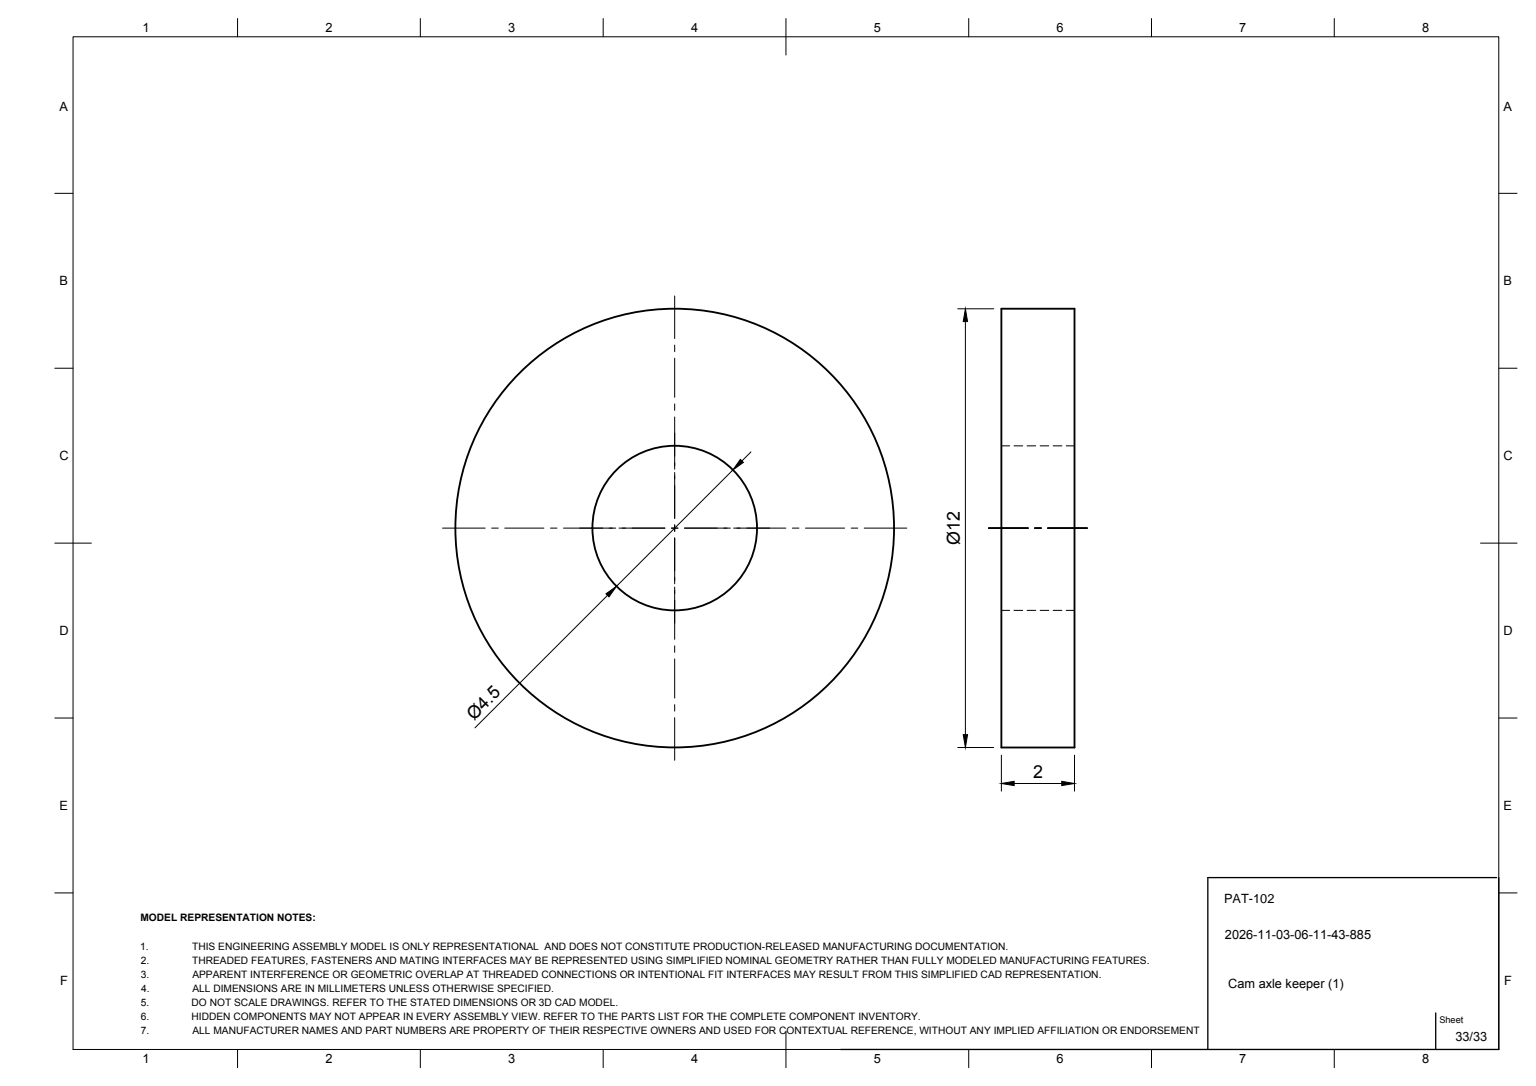
ISO-10303-21;
HEADER;
/* Generated by software containing ST-Developer
 * from STEP Tools, Inc. (www.steptools.com) 
 */

FILE_DESCRIPTION(
/* description */ ('Swing-away clamp arm'),
/* implementation_level */ '2;1');

FILE_NAME(
/* name */ 'Cam axle keeper (1).step',
/* time_stamp */ '2026-10-28T03:26:03-07:00',
/* author */ (''),
/* organization */ (''),
/* preprocessor_version */ 'ST-DEVELOPER v20.2',
/* originating_system */ 'Autodesk Translation Framework v15.17.0.0',
/* authorisation */ '');

FILE_SCHEMA (('AUTOMOTIVE_DESIGN { 1 0 10303 214 3 1 1 }'));
ENDSEC;

DATA;
#10=MECHANICAL_DESIGN_GEOMETRIC_PRESENTATION_REPRESENTATION('',(#324),#10627);
#264=SHAPE_REPRESENTATION_RELATIONSHIP('SRR','None',#10765,#290);
#290=ADVANCED_BREP_SHAPE_REPRESENTATION('',(#357),#10624);
#324=STYLED_ITEM('',(#10965),#357);
#357=MANIFOLD_SOLID_BREP('Body1',#4931);
#454=FACE_BOUND('',#1313,.T.);
#455=FACE_BOUND('',#1315,.T.);
#613=PLANE('',#5790);
#614=PLANE('',#5791);
#907=FACE_OUTER_BOUND('',#1310,.T.);
#908=FACE_OUTER_BOUND('',#1311,.T.);
#909=FACE_OUTER_BOUND('',#1312,.T.);
#910=FACE_OUTER_BOUND('',#1314,.T.);
#1310=EDGE_LOOP('',(#4361,#4362,#4363,#4364));
#1311=EDGE_LOOP('',(#4365,#4366,#4367,#4368));
#1312=EDGE_LOOP('',(#4369));
#1313=EDGE_LOOP('',(#4370));
#1314=EDGE_LOOP('',(#4371));
#1315=EDGE_LOOP('',(#4372));
#1624=LINE('',#10390,#1946);
#1625=LINE('',#10396,#1947);
#1946=VECTOR('',#7269,0.225);
#1947=VECTOR('',#7276,0.6);
#2243=CIRCLE('',#5785,0.225);
#2244=CIRCLE('',#5786,0.225);
#2245=CIRCLE('',#5788,0.6);
#2246=CIRCLE('',#5789,0.6);
#2630=VERTEX_POINT('',#10387);
#2631=VERTEX_POINT('',#10389);
#2632=VERTEX_POINT('',#10393);
#2633=VERTEX_POINT('',#10395);
#3213=EDGE_CURVE('',#2630,#2630,#2243,.T.);
#3214=EDGE_CURVE('',#2630,#2631,#1624,.T.);
#3215=EDGE_CURVE('',#2631,#2631,#2244,.T.);
#3216=EDGE_CURVE('',#2632,#2632,#2245,.T.);
#3217=EDGE_CURVE('',#2632,#2633,#1625,.T.);
#3218=EDGE_CURVE('',#2633,#2633,#2246,.T.);
#4361=ORIENTED_EDGE('',*,*,#3213,.F.);
#4362=ORIENTED_EDGE('',*,*,#3214,.T.);
#4363=ORIENTED_EDGE('',*,*,#3215,.T.);
#4364=ORIENTED_EDGE('',*,*,#3214,.F.);
#4365=ORIENTED_EDGE('',*,*,#3216,.F.);
#4366=ORIENTED_EDGE('',*,*,#3217,.T.);
#4367=ORIENTED_EDGE('',*,*,#3218,.T.);
#4368=ORIENTED_EDGE('',*,*,#3217,.F.);
#4369=ORIENTED_EDGE('',*,*,#3216,.T.);
#4370=ORIENTED_EDGE('',*,*,#3213,.T.);
#4371=ORIENTED_EDGE('',*,*,#3218,.F.);
#4372=ORIENTED_EDGE('',*,*,#3215,.F.);
#4586=CYLINDRICAL_SURFACE('',#5784,0.225);
#4587=CYLINDRICAL_SURFACE('',#5787,0.6);
#4862=ADVANCED_FACE('',(#907),#4586,.F.);
#4863=ADVANCED_FACE('',(#908),#4587,.T.);
#4864=ADVANCED_FACE('',(#909,#454),#613,.T.);
#4865=ADVANCED_FACE('',(#910,#455),#614,.F.);
#4931=CLOSED_SHELL('',(#4862,#4863,#4864,#4865));
#5783=AXIS2_PLACEMENT_3D('',#10385,#7263,#7264);
#5784=AXIS2_PLACEMENT_3D('',#10386,#7265,#7266);
#5785=AXIS2_PLACEMENT_3D('',#10388,#7267,#7268);
#5786=AXIS2_PLACEMENT_3D('',#10391,#7270,#7271);
#5787=AXIS2_PLACEMENT_3D('',#10392,#7272,#7273);
#5788=AXIS2_PLACEMENT_3D('',#10394,#7274,#7275);
#5789=AXIS2_PLACEMENT_3D('',#10397,#7277,#7278);
#5790=AXIS2_PLACEMENT_3D('',#10398,#7279,#7280);
#5791=AXIS2_PLACEMENT_3D('',#10399,#7281,#7282);
#7263=DIRECTION('axis',(0.,0.,1.));
#7264=DIRECTION('refdir',(1.,0.,0.));
#7265=DIRECTION('center_axis',(0.,1.,0.));
#7266=DIRECTION('ref_axis',(1.,0.,0.));
#7267=DIRECTION('center_axis',(0.,-1.,0.));
#7268=DIRECTION('ref_axis',(1.,0.,0.));
#7269=DIRECTION('',(0.,-1.,0.));
#7270=DIRECTION('center_axis',(0.,-1.,0.));
#7271=DIRECTION('ref_axis',(1.,0.,0.));
#7272=DIRECTION('center_axis',(0.,1.,0.));
#7273=DIRECTION('ref_axis',(1.,0.,0.));
#7274=DIRECTION('center_axis',(0.,1.,0.));
#7275=DIRECTION('ref_axis',(1.,0.,0.));
#7276=DIRECTION('',(0.,-1.,0.));
#7277=DIRECTION('center_axis',(0.,1.,0.));
#7278=DIRECTION('ref_axis',(1.,0.,0.));
#7279=DIRECTION('center_axis',(0.,1.,0.));
#7280=DIRECTION('ref_axis',(1.,0.,0.));
#7281=DIRECTION('center_axis',(0.,1.,0.));
#7282=DIRECTION('ref_axis',(1.,0.,0.));
#10385=CARTESIAN_POINT('',(0.,0.,0.));
#10386=CARTESIAN_POINT('Origin',(2.,1.8,10.5));
#10387=CARTESIAN_POINT('',(1.775,2.,10.5));
#10388=CARTESIAN_POINT('Origin',(2.,2.,10.5));
#10389=CARTESIAN_POINT('',(1.775,1.8,10.5));
#10390=CARTESIAN_POINT('',(1.775,1.8,10.5));
#10391=CARTESIAN_POINT('Origin',(2.,1.8,10.5));
#10392=CARTESIAN_POINT('Origin',(2.,1.8,10.5));
#10393=CARTESIAN_POINT('',(1.4,2.,10.5));
#10394=CARTESIAN_POINT('Origin',(2.,2.,10.5));
#10395=CARTESIAN_POINT('',(1.4,1.8,10.5));
#10396=CARTESIAN_POINT('',(1.4,1.8,10.5));
#10397=CARTESIAN_POINT('Origin',(2.,1.8,10.5));
#10398=CARTESIAN_POINT('Origin',(2.,2.,10.5));
#10399=CARTESIAN_POINT('Origin',(2.,1.8,10.5));
#10592=UNCERTAINTY_MEASURE_WITH_UNIT(LENGTH_MEASURE(0.001),#10628,
'DISTANCE_ACCURACY_VALUE',
'Maximum model space distance between geometric entities at asserted c
onnectivities');
#10595=UNCERTAINTY_MEASURE_WITH_UNIT(LENGTH_MEASURE(0.001),#10628,
'DISTANCE_ACCURACY_VALUE',
'Maximum model space distance between geometric entities at asserted c
onnectivities');
#10624=(
GEOMETRIC_REPRESENTATION_CONTEXT(3)
GLOBAL_UNCERTAINTY_ASSIGNED_CONTEXT((#10592))
GLOBAL_UNIT_ASSIGNED_CONTEXT((#10628,#10630,#10631))
REPRESENTATION_CONTEXT('','3D')
);
#10627=(
GEOMETRIC_REPRESENTATION_CONTEXT(3)
GLOBAL_UNCERTAINTY_ASSIGNED_CONTEXT((#10595))
GLOBAL_UNIT_ASSIGNED_CONTEXT((#10628,#10630,#10631))
REPRESENTATION_CONTEXT('','3D')
);
#10628=(
LENGTH_UNIT()
NAMED_UNIT(*)
SI_UNIT(.CENTI.,.METRE.)
);
#10630=(
NAMED_UNIT(*)
PLANE_ANGLE_UNIT()
SI_UNIT($,.RADIAN.)
);
#10631=(
NAMED_UNIT(*)
SI_UNIT($,.STERADIAN.)
SOLID_ANGLE_UNIT()
);
#10660=SHAPE_DEFINITION_REPRESENTATION(#10706,#10765);
#10706=PRODUCT_DEFINITION_SHAPE('',$,#10797);
#10765=SHAPE_REPRESENTATION('',(#5783),#10624);
#10768=PRODUCT_DEFINITION_CONTEXT('part definition',#10863,'design');
#10797=PRODUCT_DEFINITION('Cam axle keeper (1)','Cam axle keeper (1)',#10828,
#10768);
#10828=PRODUCT_DEFINITION_FORMATION('',$,#10893);
#10863=APPLICATION_CONTEXT(
'Core Data for Automotive Mechanical Design Process');
#10864=PRODUCT_CONTEXT('part definition',#10863,'mechanical');
#10893=PRODUCT('Cam axle keeper (1)','Cam axle keeper (1)',
'Cam axle keeper (1)',(#10864));
#10959=COLOUR_RGB('Grey',0.48,0.52,0.57);
#10960=FILL_AREA_STYLE_COLOUR('',#10959);
#10961=FILL_AREA_STYLE('',(#10960));
#10962=SURFACE_STYLE_FILL_AREA(#10961);
#10963=SURFACE_SIDE_STYLE('',(#10962));
#10964=SURFACE_STYLE_USAGE(.BOTH.,#10963);
#10965=PRESENTATION_STYLE_ASSIGNMENT((#10964));
ENDSEC;
END-ISO-10303-21;
